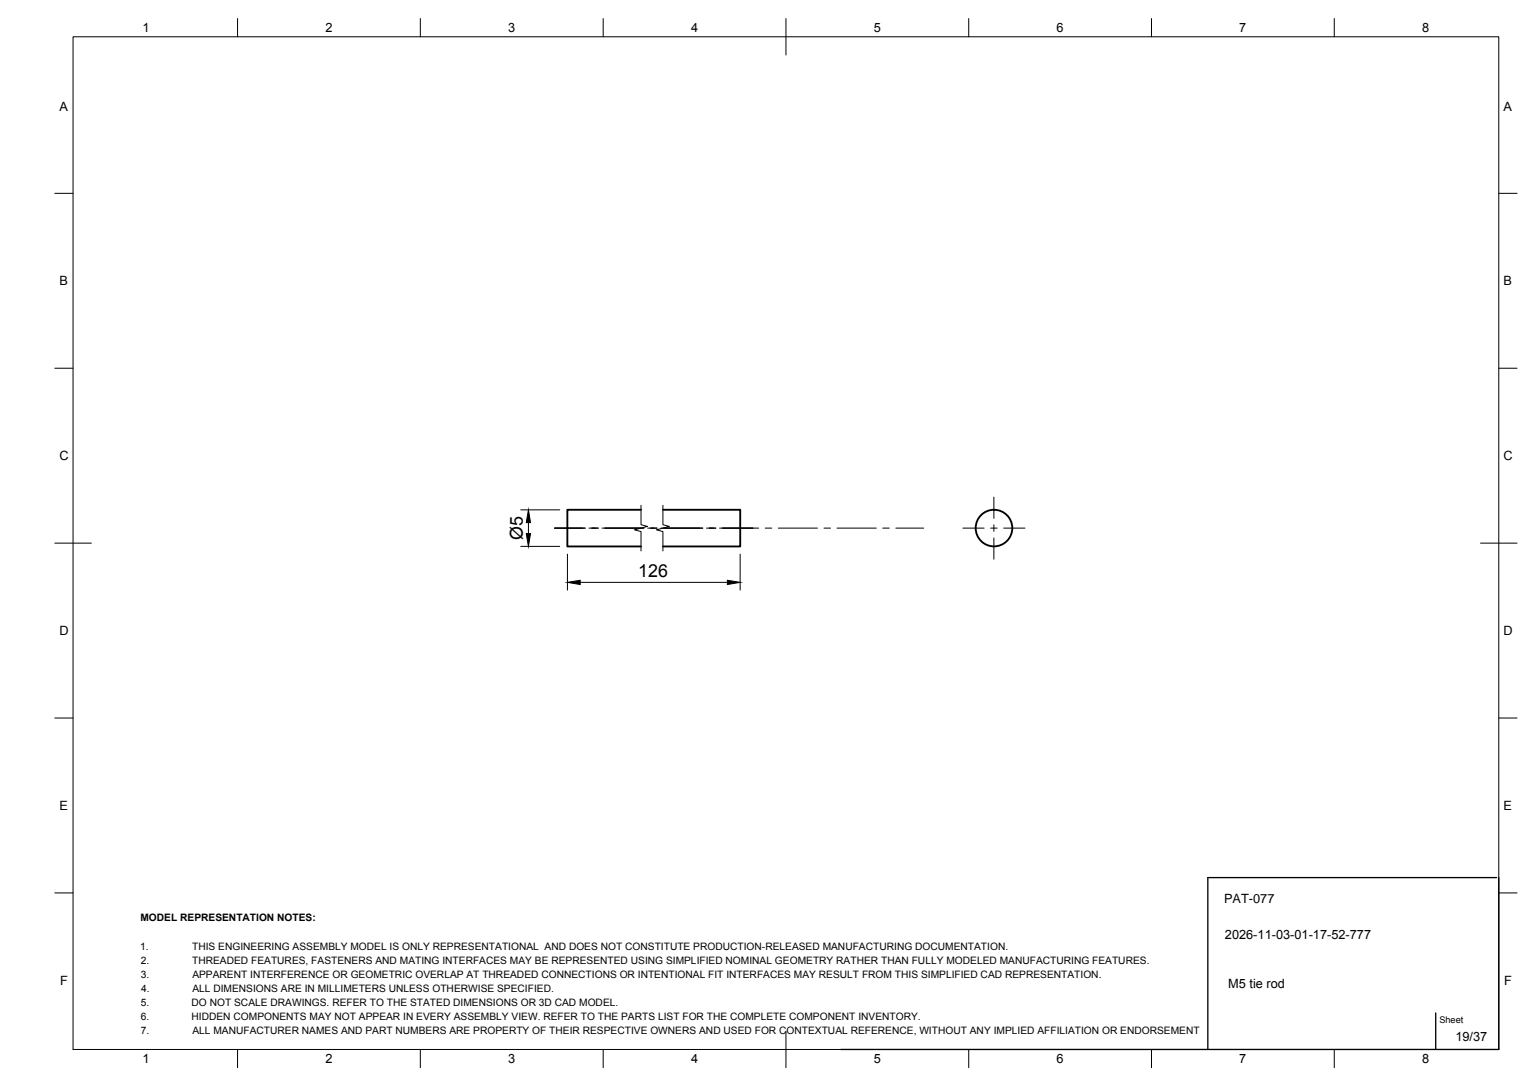
ISO-10303-21;
HEADER;
/* Generated by software containing ST-Developer
 * from STEP Tools, Inc. (www.steptools.com) 
 */

FILE_DESCRIPTION(
/* description */ ('Pallet stop with pneumatic fitting'),
/* implementation_level */ '2;1');

FILE_NAME(
/* name */ 'M5 tie rod.step',
/* time_stamp */ '2026-10-27T10:51:41-07:00',
/* author */ (''),
/* organization */ (''),
/* preprocessor_version */ 'ST-DEVELOPER v20.2',
/* originating_system */ 'Autodesk Translation Framework v15.17.0.0',
/* authorisation */ '');

FILE_SCHEMA (('AUTOMOTIVE_DESIGN { 1 0 10303 214 3 1 1 }'));
ENDSEC;

DATA;
#10=MECHANICAL_DESIGN_GEOMETRIC_PRESENTATION_REPRESENTATION('',(#371),#10265);
#307=SHAPE_REPRESENTATION_RELATIONSHIP('SRR','None',#10420,#339);
#339=ADVANCED_BREP_SHAPE_REPRESENTATION('',(#403),#10244);
#371=STYLED_ITEM('',(#10655),#403);
#403=MANIFOLD_SOLID_BREP('Body1',#5059);
#624=PLANE('',#5731);
#625=PLANE('',#5732);
#882=FACE_OUTER_BOUND('',#1281,.T.);
#883=FACE_OUTER_BOUND('',#1282,.T.);
#884=FACE_OUTER_BOUND('',#1283,.T.);
#1281=EDGE_LOOP('',(#3976,#3977,#3978,#3979));
#1282=EDGE_LOOP('',(#3980));
#1283=EDGE_LOOP('',(#3981));
#1632=LINE('',#9328,#1967);
#1967=VECTOR('',#6827,0.25);
#2294=CIRCLE('',#5729,0.25);
#2295=CIRCLE('',#5730,0.25);
#2594=VERTEX_POINT('',#9325);
#2595=VERTEX_POINT('',#9327);
#3087=EDGE_CURVE('',#2594,#2594,#2294,.T.);
#3088=EDGE_CURVE('',#2594,#2595,#1632,.T.);
#3089=EDGE_CURVE('',#2595,#2595,#2295,.T.);
#3976=ORIENTED_EDGE('',*,*,#3087,.F.);
#3977=ORIENTED_EDGE('',*,*,#3088,.T.);
#3978=ORIENTED_EDGE('',*,*,#3089,.T.);
#3979=ORIENTED_EDGE('',*,*,#3088,.F.);
#3980=ORIENTED_EDGE('',*,*,#3087,.T.);
#3981=ORIENTED_EDGE('',*,*,#3089,.F.);
#4688=CYLINDRICAL_SURFACE('',#5728,0.25);
#4877=ADVANCED_FACE('',(#882),#4688,.T.);
#4878=ADVANCED_FACE('',(#883),#624,.T.);
#4879=ADVANCED_FACE('',(#884),#625,.F.);
#5059=CLOSED_SHELL('',(#4877,#4878,#4879));
#5727=AXIS2_PLACEMENT_3D('',#9323,#6821,#6822);
#5728=AXIS2_PLACEMENT_3D('',#9324,#6823,#6824);
#5729=AXIS2_PLACEMENT_3D('',#9326,#6825,#6826);
#5730=AXIS2_PLACEMENT_3D('',#9329,#6828,#6829);
#5731=AXIS2_PLACEMENT_3D('',#9330,#6830,#6831);
#5732=AXIS2_PLACEMENT_3D('',#9331,#6832,#6833);
#6821=DIRECTION('axis',(0.,0.,1.));
#6822=DIRECTION('refdir',(1.,0.,0.));
#6823=DIRECTION('center_axis',(0.,0.,1.));
#6824=DIRECTION('ref_axis',(1.,0.,0.));
#6825=DIRECTION('center_axis',(0.,0.,1.));
#6826=DIRECTION('ref_axis',(1.,0.,0.));
#6827=DIRECTION('',(0.,0.,-1.));
#6828=DIRECTION('center_axis',(0.,0.,1.));
#6829=DIRECTION('ref_axis',(1.,0.,0.));
#6830=DIRECTION('center_axis',(0.,0.,1.));
#6831=DIRECTION('ref_axis',(1.,0.,0.));
#6832=DIRECTION('center_axis',(0.,0.,1.));
#6833=DIRECTION('ref_axis',(1.,0.,0.));
#9323=CARTESIAN_POINT('',(0.,0.,0.));
#9324=CARTESIAN_POINT('Origin',(5.27279220613579,5.27279220613579,-1.8));
#9325=CARTESIAN_POINT('',(5.02279220613579,5.27279220613579,10.8));
#9326=CARTESIAN_POINT('Origin',(5.27279220613579,5.27279220613579,10.8));
#9327=CARTESIAN_POINT('',(5.02279220613579,5.27279220613579,-1.8));
#9328=CARTESIAN_POINT('',(5.02279220613579,5.27279220613579,-1.8));
#9329=CARTESIAN_POINT('Origin',(5.27279220613579,5.27279220613579,-1.8));
#9330=CARTESIAN_POINT('Origin',(5.27279220613579,5.27279220613579,10.8));
#9331=CARTESIAN_POINT('Origin',(5.27279220613579,5.27279220613579,-1.8));
#10206=UNCERTAINTY_MEASURE_WITH_UNIT(LENGTH_MEASURE(0.001),#10266,
'DISTANCE_ACCURACY_VALUE',
'Maximum model space distance between geometric entities at asserted c
onnectivities');
#10227=UNCERTAINTY_MEASURE_WITH_UNIT(LENGTH_MEASURE(0.001),#10266,
'DISTANCE_ACCURACY_VALUE',
'Maximum model space distance between geometric entities at asserted c
onnectivities');
#10244=(
GEOMETRIC_REPRESENTATION_CONTEXT(3)
GLOBAL_UNCERTAINTY_ASSIGNED_CONTEXT((#10206))
GLOBAL_UNIT_ASSIGNED_CONTEXT((#10266,#10268,#10269))
REPRESENTATION_CONTEXT('','3D')
);
#10265=(
GEOMETRIC_REPRESENTATION_CONTEXT(3)
GLOBAL_UNCERTAINTY_ASSIGNED_CONTEXT((#10227))
GLOBAL_UNIT_ASSIGNED_CONTEXT((#10266,#10268,#10269))
REPRESENTATION_CONTEXT('','3D')
);
#10266=(
LENGTH_UNIT()
NAMED_UNIT(*)
SI_UNIT(.CENTI.,.METRE.)
);
#10268=(
NAMED_UNIT(*)
PLANE_ANGLE_UNIT()
SI_UNIT($,.RADIAN.)
);
#10269=(
NAMED_UNIT(*)
SI_UNIT($,.STERADIAN.)
SOLID_ANGLE_UNIT()
);
#10286=SHAPE_DEFINITION_REPRESENTATION(#10323,#10420);
#10323=PRODUCT_DEFINITION_SHAPE('',$,#10458);
#10420=SHAPE_REPRESENTATION('',(#5727),#10244);
#10441=PRODUCT_DEFINITION_CONTEXT('part definition',#10554,'design');
#10458=PRODUCT_DEFINITION('M5 tie rod','M5 tie rod',#10495,#10441);
#10495=PRODUCT_DEFINITION_FORMATION('',$,#10572);
#10554=APPLICATION_CONTEXT(
'Core Data for Automotive Mechanical Design Process');
#10555=PRODUCT_CONTEXT('part definition',#10554,'mechanical');
#10572=PRODUCT('M5 tie rod','M5 tie rod','M5 tie rod',(#10555));
#10649=COLOUR_RGB('Grey',0.48,0.52,0.57);
#10650=FILL_AREA_STYLE_COLOUR('',#10649);
#10651=FILL_AREA_STYLE('',(#10650));
#10652=SURFACE_STYLE_FILL_AREA(#10651);
#10653=SURFACE_SIDE_STYLE('',(#10652));
#10654=SURFACE_STYLE_USAGE(.BOTH.,#10653);
#10655=PRESENTATION_STYLE_ASSIGNMENT((#10654));
ENDSEC;
END-ISO-10303-21;
